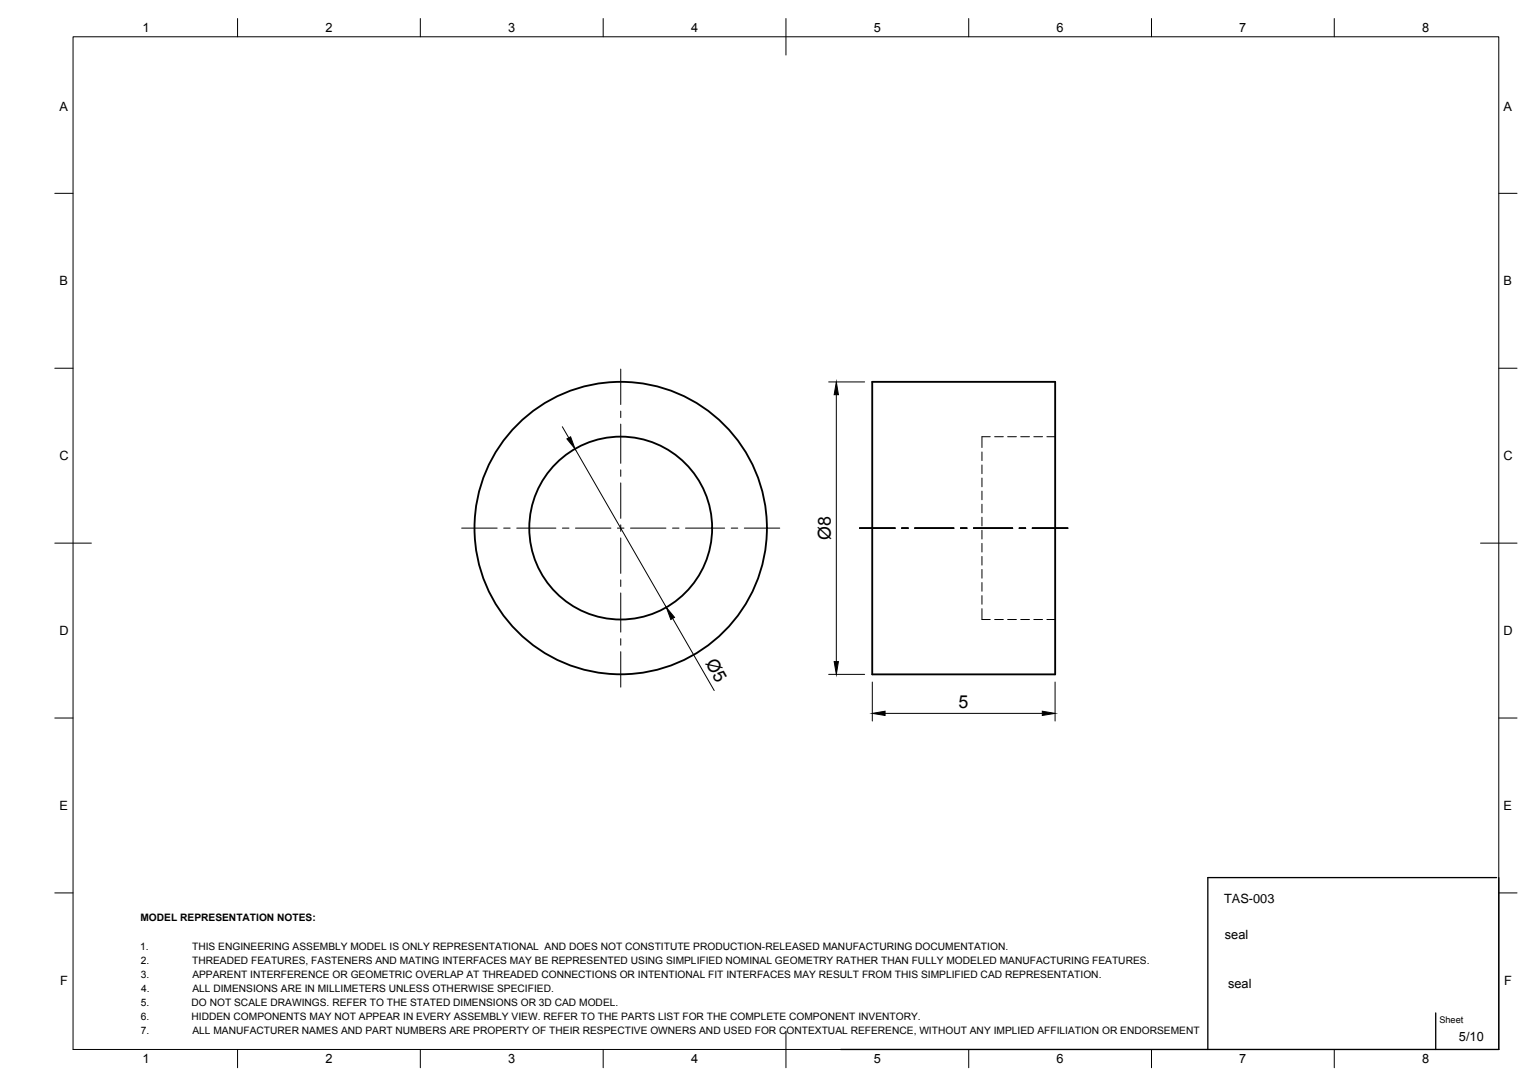
ISO-10303-21;
HEADER;
/* Generated by software containing ST-Developer
 * from STEP Tools, Inc. (www.steptools.com) 
 */

FILE_DESCRIPTION(
/* description */ ('STEP AP214'),
/* implementation_level */ '2;1');

FILE_NAME(
/* name */ 'seal.step',
/* time_stamp */ '2026-11-04T19:43:37-08:00',
/* author */ (''),
/* organization */ (''),
/* preprocessor_version */ 'ST-DEVELOPER v20.2',
/* originating_system */ 'Autodesk Translation Framework v15.17.0.0',
/* authorisation */ '');

FILE_SCHEMA (('AUTOMOTIVE_DESIGN { 1 0 10303 214 3 1 1 }'));
ENDSEC;

DATA;
#10=MECHANICAL_DESIGN_GEOMETRIC_PRESENTATION_REPRESENTATION('',(#117),#7627);
#99=SHAPE_REPRESENTATION_RELATIONSHIP('SRR','None',#7667,#108);
#108=ADVANCED_BREP_SHAPE_REPRESENTATION('',(#138),#7620);
#117=STYLED_ITEM('',(#7721),#138);
#138=MANIFOLD_SOLID_BREP('Body1',#2415);
#167=FACE_BOUND('',#504,.T.);
#205=PLANE('',#2597);
#206=PLANE('',#2598);
#207=PLANE('',#2599);
#266=CYLINDRICAL_SURFACE('',#2591,2.5);
#267=CYLINDRICAL_SURFACE('',#2594,4.);
#337=FACE_OUTER_BOUND('',#501,.T.);
#338=FACE_OUTER_BOUND('',#502,.T.);
#339=FACE_OUTER_BOUND('',#503,.T.);
#340=FACE_OUTER_BOUND('',#505,.T.);
#341=FACE_OUTER_BOUND('',#506,.T.);
#501=EDGE_LOOP('',(#1735,#1736,#1737,#1738));
#502=EDGE_LOOP('',(#1739,#1740,#1741,#1742));
#503=EDGE_LOOP('',(#1743));
#504=EDGE_LOOP('',(#1744));
#505=EDGE_LOOP('',(#1745));
#506=EDGE_LOOP('',(#1746));
#671=CIRCLE('',#2592,2.5);
#672=CIRCLE('',#2593,2.5);
#673=CIRCLE('',#2595,4.);
#674=CIRCLE('',#2596,4.);
#836=LINE('',#3812,#992);
#837=LINE('',#3818,#993);
#992=VECTOR('',#3015,2.5);
#993=VECTOR('',#3022,4.);
#1153=VERTEX_POINT('',#3809);
#1154=VERTEX_POINT('',#3811);
#1155=VERTEX_POINT('',#3815);
#1156=VERTEX_POINT('',#3817);
#1362=EDGE_CURVE('',#1153,#1153,#671,.T.);
#1363=EDGE_CURVE('',#1153,#1154,#836,.T.);
#1364=EDGE_CURVE('',#1154,#1154,#672,.T.);
#1365=EDGE_CURVE('',#1155,#1155,#673,.T.);
#1366=EDGE_CURVE('',#1155,#1156,#837,.T.);
#1367=EDGE_CURVE('',#1156,#1156,#674,.T.);
#1735=ORIENTED_EDGE('',*,*,#1362,.T.);
#1736=ORIENTED_EDGE('',*,*,#1363,.T.);
#1737=ORIENTED_EDGE('',*,*,#1364,.F.);
#1738=ORIENTED_EDGE('',*,*,#1363,.F.);
#1739=ORIENTED_EDGE('',*,*,#1365,.T.);
#1740=ORIENTED_EDGE('',*,*,#1366,.T.);
#1741=ORIENTED_EDGE('',*,*,#1367,.F.);
#1742=ORIENTED_EDGE('',*,*,#1366,.F.);
#1743=ORIENTED_EDGE('',*,*,#1365,.F.);
#1744=ORIENTED_EDGE('',*,*,#1364,.T.);
#1745=ORIENTED_EDGE('',*,*,#1362,.F.);
#1746=ORIENTED_EDGE('',*,*,#1367,.T.);
#2288=ADVANCED_FACE('',(#337),#266,.F.);
#2289=ADVANCED_FACE('',(#338),#267,.T.);
#2290=ADVANCED_FACE('',(#339,#167),#205,.F.);
#2291=ADVANCED_FACE('',(#340),#206,.F.);
#2292=ADVANCED_FACE('',(#341),#207,.T.);
#2415=CLOSED_SHELL('',(#2288,#2289,#2290,#2291,#2292));
#2590=AXIS2_PLACEMENT_3D('',#3807,#3009,#3010);
#2591=AXIS2_PLACEMENT_3D('',#3808,#3011,#3012);
#2592=AXIS2_PLACEMENT_3D('',#3810,#3013,#3014);
#2593=AXIS2_PLACEMENT_3D('',#3813,#3016,#3017);
#2594=AXIS2_PLACEMENT_3D('',#3814,#3018,#3019);
#2595=AXIS2_PLACEMENT_3D('',#3816,#3020,#3021);
#2596=AXIS2_PLACEMENT_3D('',#3819,#3023,#3024);
#2597=AXIS2_PLACEMENT_3D('',#3820,#3025,#3026);
#2598=AXIS2_PLACEMENT_3D('',#3821,#3027,#3028);
#2599=AXIS2_PLACEMENT_3D('',#3822,#3029,#3030);
#3009=DIRECTION('axis',(0.,0.,1.));
#3010=DIRECTION('refdir',(1.,0.,0.));
#3011=DIRECTION('center_axis',(0.,1.,0.));
#3012=DIRECTION('ref_axis',(0.,0.,1.));
#3013=DIRECTION('center_axis',(0.,-1.,0.));
#3014=DIRECTION('ref_axis',(0.,0.,-1.));
#3015=DIRECTION('',(0.,1.,0.));
#3016=DIRECTION('center_axis',(0.,-1.,0.));
#3017=DIRECTION('ref_axis',(0.,0.,-1.));
#3018=DIRECTION('center_axis',(0.,1.,0.));
#3019=DIRECTION('ref_axis',(0.,0.,1.));
#3020=DIRECTION('center_axis',(0.,-1.,0.));
#3021=DIRECTION('ref_axis',(0.,0.,-1.));
#3022=DIRECTION('',(0.,-1.,0.));
#3023=DIRECTION('center_axis',(0.,-1.,0.));
#3024=DIRECTION('ref_axis',(0.,0.,-1.));
#3025=DIRECTION('center_axis',(0.,-1.,0.));
#3026=DIRECTION('ref_axis',(0.,0.,-1.));
#3027=DIRECTION('center_axis',(0.,-1.,0.));
#3028=DIRECTION('ref_axis',(0.,0.,-1.));
#3029=DIRECTION('center_axis',(0.,-1.,0.));
#3030=DIRECTION('ref_axis',(0.,0.,-1.));
#3807=CARTESIAN_POINT('',(0.,0.,0.));
#3808=CARTESIAN_POINT('Origin',(0.,3.,0.));
#3809=CARTESIAN_POINT('',(-3.06161699786838E-16,3.,-2.5));
#3810=CARTESIAN_POINT('Origin',(0.,3.,0.));
#3811=CARTESIAN_POINT('',(-3.06161699786838E-16,5.,-2.5));
#3812=CARTESIAN_POINT('',(-3.06161699786838E-16,3.,-2.5));
#3813=CARTESIAN_POINT('Origin',(0.,5.,0.));
#3814=CARTESIAN_POINT('Origin',(0.,3.,0.));
#3815=CARTESIAN_POINT('',(-4.89858719658941E-16,5.,-4.));
#3816=CARTESIAN_POINT('Origin',(0.,5.,0.));
#3817=CARTESIAN_POINT('',(-4.89858719658941E-16,0.,-4.));
#3818=CARTESIAN_POINT('',(-4.89858719658941E-16,3.,-4.));
#3819=CARTESIAN_POINT('Origin',(0.,0.,0.));
#3820=CARTESIAN_POINT('Origin',(0.,5.,0.));
#3821=CARTESIAN_POINT('Origin',(0.,3.,0.));
#3822=CARTESIAN_POINT('Origin',(0.,0.,0.));
#7609=UNCERTAINTY_MEASURE_WITH_UNIT(LENGTH_MEASURE(0.01),#7628,
'DISTANCE_ACCURACY_VALUE',
'Maximum model space distance between geometric entities at asserted c
onnectivities');
#7616=UNCERTAINTY_MEASURE_WITH_UNIT(LENGTH_MEASURE(0.01),#7628,
'DISTANCE_ACCURACY_VALUE',
'Maximum model space distance between geometric entities at asserted c
onnectivities');
#7620=(
GEOMETRIC_REPRESENTATION_CONTEXT(3)
GLOBAL_UNCERTAINTY_ASSIGNED_CONTEXT((#7609))
GLOBAL_UNIT_ASSIGNED_CONTEXT((#7628,#7630,#7631))
REPRESENTATION_CONTEXT('','3D')
);
#7627=(
GEOMETRIC_REPRESENTATION_CONTEXT(3)
GLOBAL_UNCERTAINTY_ASSIGNED_CONTEXT((#7616))
GLOBAL_UNIT_ASSIGNED_CONTEXT((#7628,#7630,#7631))
REPRESENTATION_CONTEXT('','3D')
);
#7628=(
LENGTH_UNIT()
NAMED_UNIT(*)
SI_UNIT(.MILLI.,.METRE.)
);
#7630=(
NAMED_UNIT(*)
PLANE_ANGLE_UNIT()
SI_UNIT($,.RADIAN.)
);
#7631=(
NAMED_UNIT(*)
SI_UNIT($,.STERADIAN.)
SOLID_ANGLE_UNIT()
);
#7635=SHAPE_DEFINITION_REPRESENTATION(#7645,#7667);
#7645=PRODUCT_DEFINITION_SHAPE('',$,#7678);
#7667=SHAPE_REPRESENTATION('',(#2590),#7620);
#7674=PRODUCT_DEFINITION_CONTEXT('part definition',#7706,'design');
#7678=PRODUCT_DEFINITION('seal','seal',#7688,#7674);
#7688=PRODUCT_DEFINITION_FORMATION('',$,#7711);
#7706=APPLICATION_CONTEXT(
'Core Data for Automotive Mechanical Design Process');
#7707=PRODUCT_CONTEXT('part definition',#7706,'mechanical');
#7711=PRODUCT('seal','seal',$,(#7707));
#7721=PRESENTATION_STYLE_ASSIGNMENT((#7727));
#7727=SURFACE_STYLE_USAGE(.BOTH.,#7733);
#7733=SURFACE_SIDE_STYLE('',(#7739));
#7739=SURFACE_STYLE_FILL_AREA(#7745);
#7745=FILL_AREA_STYLE('Opaque(31,36,43)',(#7751));
#7751=FILL_AREA_STYLE_COLOUR('Opaque(31,36,43)',#7757);
#7757=COLOUR_RGB('Opaque(31,36,43)',0.12156862745098,0.141176470588235,
0.168627450980392);
ENDSEC;
END-ISO-10303-21;
